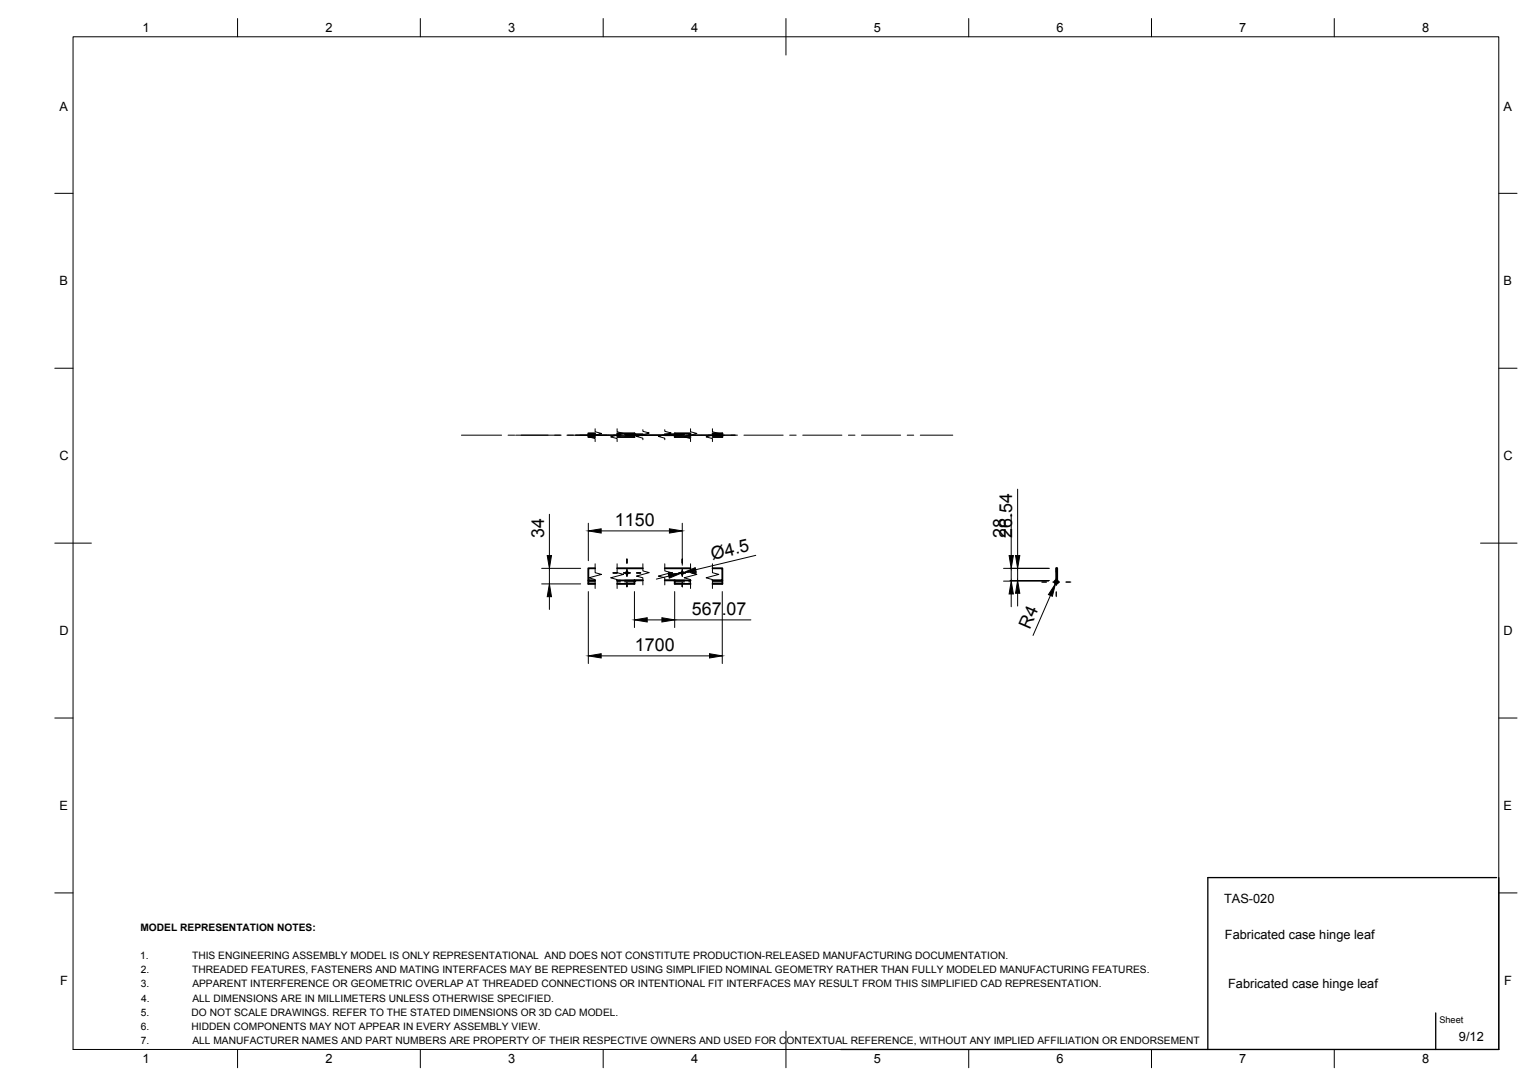
ISO-10303-21;
HEADER;
/* Generated by software containing ST-Developer
 * from STEP Tools, Inc. (www.steptools.com) 
 */

FILE_DESCRIPTION(
/* description */ (''),
/* implementation_level */ '2;1');

FILE_NAME(
/* name */ 'Fabricated case hinge leaf.step',
/* time_stamp */ '2026-11-15T17:46:57-08:00',
/* author */ (''),
/* organization */ (''),
/* preprocessor_version */ 'ST-DEVELOPER v20.2',
/* originating_system */ 'Autodesk Translation Framework v15.17.0.0',
/* authorisation */ '');

FILE_SCHEMA (('AUTOMOTIVE_DESIGN { 1 0 10303 214 3 1 1 }'));
ENDSEC;

DATA;
#10=MECHANICAL_DESIGN_GEOMETRIC_PRESENTATION_REPRESENTATION('',(#381),#12963);
#357=SHAPE_REPRESENTATION_RELATIONSHIP('SRR','None',#13041,#369);
#369=ADVANCED_BREP_SHAPE_REPRESENTATION('',(#393),#12957);
#381=STYLED_ITEM('',(#13110),#393);
#393=MANIFOLD_SOLID_BREP('Body1',#4815);
#423=FACE_BOUND('',#962,.T.);
#424=FACE_BOUND('',#963,.T.);
#425=FACE_BOUND('',#970,.T.);
#426=FACE_BOUND('',#972,.T.);
#427=FACE_BOUND('',#973,.T.);
#428=FACE_BOUND('',#979,.T.);
#527=PLANE('',#5108);
#528=PLANE('',#5112);
#529=PLANE('',#5113);
#530=PLANE('',#5114);
#531=PLANE('',#5115);
#532=PLANE('',#5116);
#533=PLANE('',#5123);
#534=PLANE('',#5124);
#535=PLANE('',#5131);
#536=PLANE('',#5132);
#537=PLANE('',#5133);
#676=FACE_OUTER_BOUND('',#956,.T.);
#677=FACE_OUTER_BOUND('',#957,.T.);
#678=FACE_OUTER_BOUND('',#958,.T.);
#679=FACE_OUTER_BOUND('',#959,.T.);
#680=FACE_OUTER_BOUND('',#960,.T.);
#681=FACE_OUTER_BOUND('',#961,.T.);
#682=FACE_OUTER_BOUND('',#964,.T.);
#683=FACE_OUTER_BOUND('',#965,.T.);
#684=FACE_OUTER_BOUND('',#966,.T.);
#685=FACE_OUTER_BOUND('',#967,.T.);
#686=FACE_OUTER_BOUND('',#968,.T.);
#687=FACE_OUTER_BOUND('',#969,.T.);
#688=FACE_OUTER_BOUND('',#971,.T.);
#689=FACE_OUTER_BOUND('',#974,.T.);
#690=FACE_OUTER_BOUND('',#975,.T.);
#691=FACE_OUTER_BOUND('',#976,.T.);
#692=FACE_OUTER_BOUND('',#977,.T.);
#693=FACE_OUTER_BOUND('',#978,.T.);
#956=EDGE_LOOP('',(#3604,#3605,#3606,#3607));
#957=EDGE_LOOP('',(#3608,#3609,#3610,#3611));
#958=EDGE_LOOP('',(#3612,#3613,#3614,#3615));
#959=EDGE_LOOP('',(#3616,#3617,#3618,#3619));
#960=EDGE_LOOP('',(#3620,#3621,#3622,#3623));
#961=EDGE_LOOP('',(#3624,#3625,#3626,#3627,#3628,#3629,#3630,#3631,#3632,
#3633,#3634,#3635));
#962=EDGE_LOOP('',(#3636));
#963=EDGE_LOOP('',(#3637));
#964=EDGE_LOOP('',(#3638,#3639,#3640,#3641,#3642,#3643));
#965=EDGE_LOOP('',(#3644,#3645,#3646,#3647,#3648,#3649));
#966=EDGE_LOOP('',(#3650,#3651,#3652,#3653,#3654));
#967=EDGE_LOOP('',(#3655,#3656,#3657,#3658));
#968=EDGE_LOOP('',(#3659,#3660,#3661,#3662));
#969=EDGE_LOOP('',(#3663,#3664,#3665,#3666));
#970=EDGE_LOOP('',(#3667,#3668,#3669));
#971=EDGE_LOOP('',(#3670,#3671,#3672,#3673,#3674,#3675,#3676,#3677,#3678,
#3679,#3680,#3681,#3682,#3683,#3684,#3685));
#972=EDGE_LOOP('',(#3686));
#973=EDGE_LOOP('',(#3687));
#974=EDGE_LOOP('',(#3688,#3689,#3690,#3691));
#975=EDGE_LOOP('',(#3692,#3693,#3694,#3695));
#976=EDGE_LOOP('',(#3696,#3697,#3698,#3699,#3700));
#977=EDGE_LOOP('',(#3701,#3702,#3703,#3704));
#978=EDGE_LOOP('',(#3705,#3706,#3707,#3708));
#979=EDGE_LOOP('',(#3709,#3710,#3711));
#1336=LINE('',#7043,#1738);
#1337=LINE('',#7049,#1739);
#1338=LINE('',#7054,#1740);
#1339=LINE('',#7058,#1741);
#1340=LINE('',#7059,#1742);
#1341=LINE('',#7062,#1743);
#1342=LINE('',#7065,#1744);
#1343=LINE('',#7068,#1745);
#1344=LINE('',#7070,#1746);
#1345=LINE('',#7071,#1747);
#1346=LINE('',#7074,#1748);
#1347=LINE('',#7076,#1749);
#1348=LINE('',#7078,#1750);
#1349=LINE('',#7080,#1751);
#1350=LINE('',#7082,#1752);
#1351=LINE('',#7084,#1753);
#1352=LINE('',#7086,#1754);
#1353=LINE('',#7088,#1755);
#1354=LINE('',#7089,#1756);
#1355=LINE('',#7092,#1757);
#1356=LINE('',#7094,#1758);
#1357=LINE('',#7096,#1759);
#1358=LINE('',#7097,#1760);
#1359=LINE('',#7100,#1761);
#1360=LINE('',#7102,#1762);
#1361=LINE('',#7104,#1763);
#1362=LINE('',#7105,#1764);
#1363=LINE('',#7110,#1765);
#1364=LINE('',#7115,#1766);
#1365=LINE('',#7118,#1767);
#1366=LINE('',#7122,#1768);
#1367=LINE('',#7123,#1769);
#1368=LINE('',#7124,#1770);
#1369=LINE('',#7127,#1771);
#1370=LINE('',#7129,#1772);
#1371=LINE('',#7131,#1773);
#1372=LINE('',#7133,#1774);
#1373=LINE('',#7135,#1775);
#1374=LINE('',#7136,#1776);
#1375=LINE('',#7145,#1777);
#1738=VECTOR('',#5851,0.225000000000001);
#1739=VECTOR('',#5858,0.224999999999994);
#1740=VECTOR('',#5863,1.);
#1741=VECTOR('',#5866,1.);
#1742=VECTOR('',#5867,1.);
#1743=VECTOR('',#5870,1.);
#1744=VECTOR('',#5873,1.);
#1745=VECTOR('',#5876,1.);
#1746=VECTOR('',#5877,1.);
#1747=VECTOR('',#5878,1.);
#1748=VECTOR('',#5881,1.);
#1749=VECTOR('',#5882,1.);
#1750=VECTOR('',#5883,1.);
#1751=VECTOR('',#5884,1.);
#1752=VECTOR('',#5885,1.);
#1753=VECTOR('',#5886,1.);
#1754=VECTOR('',#5887,1.);
#1755=VECTOR('',#5888,1.);
#1756=VECTOR('',#5889,1.);
#1757=VECTOR('',#5892,1.);
#1758=VECTOR('',#5893,1.);
#1759=VECTOR('',#5894,1.);
#1760=VECTOR('',#5895,1.);
#1761=VECTOR('',#5898,1.);
#1762=VECTOR('',#5899,1.);
#1763=VECTOR('',#5900,1.);
#1764=VECTOR('',#5901,1.);
#1765=VECTOR('',#5906,1.);
#1766=VECTOR('',#5913,1.);
#1767=VECTOR('',#5916,1.);
#1768=VECTOR('',#5921,1.);
#1769=VECTOR('',#5922,1.);
#1770=VECTOR('',#5923,1.);
#1771=VECTOR('',#5926,1.);
#1772=VECTOR('',#5927,1.);
#1773=VECTOR('',#5928,1.);
#1774=VECTOR('',#5929,1.);
#1775=VECTOR('',#5930,1.);
#1776=VECTOR('',#5931,1.);
#1777=VECTOR('',#5948,1.);
#1966=CIRCLE('',#5103,0.225000000000001);
#1967=CIRCLE('',#5104,0.225000000000001);
#1968=CIRCLE('',#5106,0.224999999999994);
#1969=CIRCLE('',#5107,0.224999999999994);
#1970=CIRCLE('',#5109,0.42);
#1971=CIRCLE('',#5111,0.42);
#1972=CIRCLE('',#5117,0.4);
#1973=CIRCLE('',#5118,0.22);
#1974=CIRCLE('',#5120,0.4);
#1975=CIRCLE('',#5122,0.22);
#1976=CIRCLE('',#5126,0.22);
#1977=CIRCLE('',#5127,0.22);
#1978=CIRCLE('',#5129,0.4);
#1979=CIRCLE('',#5130,0.4);
#2176=VERTEX_POINT('',#7040);
#2177=VERTEX_POINT('',#7042);
#2178=VERTEX_POINT('',#7046);
#2179=VERTEX_POINT('',#7048);
#2180=VERTEX_POINT('',#7052);
#2181=VERTEX_POINT('',#7053);
#2182=VERTEX_POINT('',#7055);
#2183=VERTEX_POINT('',#7057);
#2184=VERTEX_POINT('',#7061);
#2185=VERTEX_POINT('',#7063);
#2186=VERTEX_POINT('',#7067);
#2187=VERTEX_POINT('',#7069);
#2188=VERTEX_POINT('',#7073);
#2189=VERTEX_POINT('',#7075);
#2190=VERTEX_POINT('',#7077);
#2191=VERTEX_POINT('',#7079);
#2192=VERTEX_POINT('',#7081);
#2193=VERTEX_POINT('',#7083);
#2194=VERTEX_POINT('',#7085);
#2195=VERTEX_POINT('',#7087);
#2196=VERTEX_POINT('',#7091);
#2197=VERTEX_POINT('',#7093);
#2198=VERTEX_POINT('',#7095);
#2199=VERTEX_POINT('',#7099);
#2200=VERTEX_POINT('',#7101);
#2201=VERTEX_POINT('',#7103);
#2202=VERTEX_POINT('',#7107);
#2203=VERTEX_POINT('',#7109);
#2204=VERTEX_POINT('',#7113);
#2205=VERTEX_POINT('',#7117);
#2206=VERTEX_POINT('',#7121);
#2207=VERTEX_POINT('',#7126);
#2208=VERTEX_POINT('',#7128);
#2209=VERTEX_POINT('',#7130);
#2210=VERTEX_POINT('',#7132);
#2211=VERTEX_POINT('',#7134);
#2698=EDGE_CURVE('',#2176,#2176,#1966,.T.);
#2699=EDGE_CURVE('',#2176,#2177,#1336,.T.);
#2700=EDGE_CURVE('',#2177,#2177,#1967,.T.);
#2701=EDGE_CURVE('',#2178,#2178,#1968,.T.);
#2702=EDGE_CURVE('',#2178,#2179,#1337,.T.);
#2703=EDGE_CURVE('',#2179,#2179,#1969,.T.);
#2704=EDGE_CURVE('',#2180,#2181,#1338,.T.);
#2705=EDGE_CURVE('',#2182,#2180,#1970,.T.);
#2706=EDGE_CURVE('',#2183,#2182,#1339,.T.);
#2707=EDGE_CURVE('',#2181,#2183,#1340,.T.);
#2708=EDGE_CURVE('',#2184,#2180,#1341,.T.);
#2709=EDGE_CURVE('',#2185,#2184,#1971,.T.);
#2710=EDGE_CURVE('',#2182,#2185,#1342,.T.);
#2711=EDGE_CURVE('',#2186,#2184,#1343,.T.);
#2712=EDGE_CURVE('',#2187,#2186,#1344,.T.);
#2713=EDGE_CURVE('',#2185,#2187,#1345,.T.);
#2714=EDGE_CURVE('',#2188,#2187,#1346,.T.);
#2715=EDGE_CURVE('',#2188,#2189,#1347,.T.);
#2716=EDGE_CURVE('',#2189,#2190,#1348,.T.);
#2717=EDGE_CURVE('',#2190,#2191,#1349,.T.);
#2718=EDGE_CURVE('',#2191,#2192,#1350,.T.);
#2719=EDGE_CURVE('',#2193,#2192,#1351,.T.);
#2720=EDGE_CURVE('',#2193,#2194,#1352,.T.);
#2721=EDGE_CURVE('',#2194,#2195,#1353,.T.);
#2722=EDGE_CURVE('',#2183,#2195,#1354,.T.);
#2723=EDGE_CURVE('',#2196,#2186,#1355,.T.);
#2724=EDGE_CURVE('',#2196,#2197,#1356,.T.);
#2725=EDGE_CURVE('',#2197,#2198,#1357,.T.);
#2726=EDGE_CURVE('',#2198,#2188,#1358,.T.);
#2727=EDGE_CURVE('',#2195,#2199,#1359,.T.);
#2728=EDGE_CURVE('',#2199,#2200,#1360,.T.);
#2729=EDGE_CURVE('',#2201,#2200,#1361,.T.);
#2730=EDGE_CURVE('',#2181,#2201,#1362,.T.);
#2731=EDGE_CURVE('',#2202,#2194,#1972,.T.);
#2732=EDGE_CURVE('',#2203,#2202,#1363,.T.);
#2733=EDGE_CURVE('',#2199,#2203,#1973,.T.);
#2734=EDGE_CURVE('',#2204,#2193,#1974,.T.);
#2735=EDGE_CURVE('',#2202,#2204,#1364,.T.);
#2736=EDGE_CURVE('',#2205,#2203,#1365,.T.);
#2737=EDGE_CURVE('',#2200,#2205,#1975,.T.);
#2738=EDGE_CURVE('',#2192,#2206,#1366,.T.);
#2739=EDGE_CURVE('',#2206,#2204,#1367,.T.);
#2740=EDGE_CURVE('',#2205,#2201,#1368,.T.);
#2741=EDGE_CURVE('',#2207,#2206,#1369,.T.);
#2742=EDGE_CURVE('',#2207,#2208,#1370,.T.);
#2743=EDGE_CURVE('',#2208,#2209,#1371,.T.);
#2744=EDGE_CURVE('',#2209,#2210,#1372,.T.);
#2745=EDGE_CURVE('',#2210,#2211,#1373,.T.);
#2746=EDGE_CURVE('',#2211,#2196,#1374,.T.);
#2747=EDGE_CURVE('',#2197,#2211,#1976,.T.);
#2748=EDGE_CURVE('',#2198,#2210,#1977,.T.);
#2749=EDGE_CURVE('',#2209,#2189,#1978,.T.);
#2750=EDGE_CURVE('',#2208,#2190,#1979,.T.);
#2751=EDGE_CURVE('',#2191,#2207,#1375,.T.);
#3604=ORIENTED_EDGE('',*,*,#2698,.F.);
#3605=ORIENTED_EDGE('',*,*,#2699,.T.);
#3606=ORIENTED_EDGE('',*,*,#2700,.F.);
#3607=ORIENTED_EDGE('',*,*,#2699,.F.);
#3608=ORIENTED_EDGE('',*,*,#2701,.F.);
#3609=ORIENTED_EDGE('',*,*,#2702,.T.);
#3610=ORIENTED_EDGE('',*,*,#2703,.F.);
#3611=ORIENTED_EDGE('',*,*,#2702,.F.);
#3612=ORIENTED_EDGE('',*,*,#2704,.F.);
#3613=ORIENTED_EDGE('',*,*,#2705,.F.);
#3614=ORIENTED_EDGE('',*,*,#2706,.F.);
#3615=ORIENTED_EDGE('',*,*,#2707,.F.);
#3616=ORIENTED_EDGE('',*,*,#2708,.F.);
#3617=ORIENTED_EDGE('',*,*,#2709,.F.);
#3618=ORIENTED_EDGE('',*,*,#2710,.F.);
#3619=ORIENTED_EDGE('',*,*,#2705,.T.);
#3620=ORIENTED_EDGE('',*,*,#2711,.F.);
#3621=ORIENTED_EDGE('',*,*,#2712,.F.);
#3622=ORIENTED_EDGE('',*,*,#2713,.F.);
#3623=ORIENTED_EDGE('',*,*,#2709,.T.);
#3624=ORIENTED_EDGE('',*,*,#2706,.T.);
#3625=ORIENTED_EDGE('',*,*,#2710,.T.);
#3626=ORIENTED_EDGE('',*,*,#2713,.T.);
#3627=ORIENTED_EDGE('',*,*,#2714,.F.);
#3628=ORIENTED_EDGE('',*,*,#2715,.T.);
#3629=ORIENTED_EDGE('',*,*,#2716,.T.);
#3630=ORIENTED_EDGE('',*,*,#2717,.T.);
#3631=ORIENTED_EDGE('',*,*,#2718,.T.);
#3632=ORIENTED_EDGE('',*,*,#2719,.F.);
#3633=ORIENTED_EDGE('',*,*,#2720,.T.);
#3634=ORIENTED_EDGE('',*,*,#2721,.T.);
#3635=ORIENTED_EDGE('',*,*,#2722,.F.);
#3636=ORIENTED_EDGE('',*,*,#2700,.T.);
#3637=ORIENTED_EDGE('',*,*,#2703,.T.);
#3638=ORIENTED_EDGE('',*,*,#2712,.T.);
#3639=ORIENTED_EDGE('',*,*,#2723,.F.);
#3640=ORIENTED_EDGE('',*,*,#2724,.T.);
#3641=ORIENTED_EDGE('',*,*,#2725,.T.);
#3642=ORIENTED_EDGE('',*,*,#2726,.T.);
#3643=ORIENTED_EDGE('',*,*,#2714,.T.);
#3644=ORIENTED_EDGE('',*,*,#2707,.T.);
#3645=ORIENTED_EDGE('',*,*,#2722,.T.);
#3646=ORIENTED_EDGE('',*,*,#2727,.T.);
#3647=ORIENTED_EDGE('',*,*,#2728,.T.);
#3648=ORIENTED_EDGE('',*,*,#2729,.F.);
#3649=ORIENTED_EDGE('',*,*,#2730,.F.);
#3650=ORIENTED_EDGE('',*,*,#2727,.F.);
#3651=ORIENTED_EDGE('',*,*,#2721,.F.);
#3652=ORIENTED_EDGE('',*,*,#2731,.F.);
#3653=ORIENTED_EDGE('',*,*,#2732,.F.);
#3654=ORIENTED_EDGE('',*,*,#2733,.F.);
#3655=ORIENTED_EDGE('',*,*,#2720,.F.);
#3656=ORIENTED_EDGE('',*,*,#2734,.F.);
#3657=ORIENTED_EDGE('',*,*,#2735,.F.);
#3658=ORIENTED_EDGE('',*,*,#2731,.T.);
#3659=ORIENTED_EDGE('',*,*,#2728,.F.);
#3660=ORIENTED_EDGE('',*,*,#2733,.T.);
#3661=ORIENTED_EDGE('',*,*,#2736,.F.);
#3662=ORIENTED_EDGE('',*,*,#2737,.F.);
#3663=ORIENTED_EDGE('',*,*,#2719,.T.);
#3664=ORIENTED_EDGE('',*,*,#2738,.T.);
#3665=ORIENTED_EDGE('',*,*,#2739,.T.);
#3666=ORIENTED_EDGE('',*,*,#2734,.T.);
#3667=ORIENTED_EDGE('',*,*,#2737,.T.);
#3668=ORIENTED_EDGE('',*,*,#2740,.T.);
#3669=ORIENTED_EDGE('',*,*,#2729,.T.);
#3670=ORIENTED_EDGE('',*,*,#2704,.T.);
#3671=ORIENTED_EDGE('',*,*,#2730,.T.);
#3672=ORIENTED_EDGE('',*,*,#2740,.F.);
#3673=ORIENTED_EDGE('',*,*,#2736,.T.);
#3674=ORIENTED_EDGE('',*,*,#2732,.T.);
#3675=ORIENTED_EDGE('',*,*,#2735,.T.);
#3676=ORIENTED_EDGE('',*,*,#2739,.F.);
#3677=ORIENTED_EDGE('',*,*,#2741,.F.);
#3678=ORIENTED_EDGE('',*,*,#2742,.T.);
#3679=ORIENTED_EDGE('',*,*,#2743,.T.);
#3680=ORIENTED_EDGE('',*,*,#2744,.T.);
#3681=ORIENTED_EDGE('',*,*,#2745,.T.);
#3682=ORIENTED_EDGE('',*,*,#2746,.T.);
#3683=ORIENTED_EDGE('',*,*,#2723,.T.);
#3684=ORIENTED_EDGE('',*,*,#2711,.T.);
#3685=ORIENTED_EDGE('',*,*,#2708,.T.);
#3686=ORIENTED_EDGE('',*,*,#2698,.T.);
#3687=ORIENTED_EDGE('',*,*,#2701,.T.);
#3688=ORIENTED_EDGE('',*,*,#2725,.F.);
#3689=ORIENTED_EDGE('',*,*,#2747,.T.);
#3690=ORIENTED_EDGE('',*,*,#2745,.F.);
#3691=ORIENTED_EDGE('',*,*,#2748,.F.);
#3692=ORIENTED_EDGE('',*,*,#2716,.F.);
#3693=ORIENTED_EDGE('',*,*,#2749,.F.);
#3694=ORIENTED_EDGE('',*,*,#2743,.F.);
#3695=ORIENTED_EDGE('',*,*,#2750,.T.);
#3696=ORIENTED_EDGE('',*,*,#2726,.F.);
#3697=ORIENTED_EDGE('',*,*,#2748,.T.);
#3698=ORIENTED_EDGE('',*,*,#2744,.F.);
#3699=ORIENTED_EDGE('',*,*,#2749,.T.);
#3700=ORIENTED_EDGE('',*,*,#2715,.F.);
#3701=ORIENTED_EDGE('',*,*,#2751,.T.);
#3702=ORIENTED_EDGE('',*,*,#2741,.T.);
#3703=ORIENTED_EDGE('',*,*,#2738,.F.);
#3704=ORIENTED_EDGE('',*,*,#2718,.F.);
#3705=ORIENTED_EDGE('',*,*,#2750,.F.);
#3706=ORIENTED_EDGE('',*,*,#2742,.F.);
#3707=ORIENTED_EDGE('',*,*,#2751,.F.);
#3708=ORIENTED_EDGE('',*,*,#2717,.F.);
#3709=ORIENTED_EDGE('',*,*,#2724,.F.);
#3710=ORIENTED_EDGE('',*,*,#2746,.F.);
#3711=ORIENTED_EDGE('',*,*,#2747,.F.);
#4450=CYLINDRICAL_SURFACE('',#5102,0.225000000000001);
#4451=CYLINDRICAL_SURFACE('',#5105,0.224999999999994);
#4452=CYLINDRICAL_SURFACE('',#5110,0.42);
#4453=CYLINDRICAL_SURFACE('',#5119,0.4);
#4454=CYLINDRICAL_SURFACE('',#5121,0.22);
#4455=CYLINDRICAL_SURFACE('',#5125,0.22);
#4456=CYLINDRICAL_SURFACE('',#5128,0.4);
#4657=ADVANCED_FACE('',(#676),#4450,.F.);
#4658=ADVANCED_FACE('',(#677),#4451,.F.);
#4659=ADVANCED_FACE('',(#678),#527,.F.);
#4660=ADVANCED_FACE('',(#679),#4452,.F.);
#4661=ADVANCED_FACE('',(#680),#528,.T.);
#4662=ADVANCED_FACE('',(#681,#423,#424),#529,.T.);
#4663=ADVANCED_FACE('',(#682),#530,.T.);
#4664=ADVANCED_FACE('',(#683),#531,.T.);
#4665=ADVANCED_FACE('',(#684),#532,.F.);
#4666=ADVANCED_FACE('',(#685),#4453,.T.);
#4667=ADVANCED_FACE('',(#686),#4454,.F.);
#4668=ADVANCED_FACE('',(#687,#425),#533,.T.);
#4669=ADVANCED_FACE('',(#688,#426,#427),#534,.T.);
#4670=ADVANCED_FACE('',(#689),#4455,.F.);
#4671=ADVANCED_FACE('',(#690),#4456,.T.);
#4672=ADVANCED_FACE('',(#691),#535,.T.);
#4673=ADVANCED_FACE('',(#692),#536,.T.);
#4674=ADVANCED_FACE('',(#693,#428),#537,.F.);
#4815=CLOSED_SHELL('',(#4657,#4658,#4659,#4660,#4661,#4662,#4663,#4664,
#4665,#4666,#4667,#4668,#4669,#4670,#4671,#4672,#4673,#4674));
#5101=AXIS2_PLACEMENT_3D('',#7038,#5845,#5846);
#5102=AXIS2_PLACEMENT_3D('',#7039,#5847,#5848);
#5103=AXIS2_PLACEMENT_3D('',#7041,#5849,#5850);
#5104=AXIS2_PLACEMENT_3D('',#7044,#5852,#5853);
#5105=AXIS2_PLACEMENT_3D('',#7045,#5854,#5855);
#5106=AXIS2_PLACEMENT_3D('',#7047,#5856,#5857);
#5107=AXIS2_PLACEMENT_3D('',#7050,#5859,#5860);
#5108=AXIS2_PLACEMENT_3D('',#7051,#5861,#5862);
#5109=AXIS2_PLACEMENT_3D('',#7056,#5864,#5865);
#5110=AXIS2_PLACEMENT_3D('',#7060,#5868,#5869);
#5111=AXIS2_PLACEMENT_3D('',#7064,#5871,#5872);
#5112=AXIS2_PLACEMENT_3D('',#7066,#5874,#5875);
#5113=AXIS2_PLACEMENT_3D('',#7072,#5879,#5880);
#5114=AXIS2_PLACEMENT_3D('',#7090,#5890,#5891);
#5115=AXIS2_PLACEMENT_3D('',#7098,#5896,#5897);
#5116=AXIS2_PLACEMENT_3D('',#7106,#5902,#5903);
#5117=AXIS2_PLACEMENT_3D('',#7108,#5904,#5905);
#5118=AXIS2_PLACEMENT_3D('',#7111,#5907,#5908);
#5119=AXIS2_PLACEMENT_3D('',#7112,#5909,#5910);
#5120=AXIS2_PLACEMENT_3D('',#7114,#5911,#5912);
#5121=AXIS2_PLACEMENT_3D('',#7116,#5914,#5915);
#5122=AXIS2_PLACEMENT_3D('',#7119,#5917,#5918);
#5123=AXIS2_PLACEMENT_3D('',#7120,#5919,#5920);
#5124=AXIS2_PLACEMENT_3D('',#7125,#5924,#5925);
#5125=AXIS2_PLACEMENT_3D('',#7137,#5932,#5933);
#5126=AXIS2_PLACEMENT_3D('',#7138,#5934,#5935);
#5127=AXIS2_PLACEMENT_3D('',#7139,#5936,#5937);
#5128=AXIS2_PLACEMENT_3D('',#7140,#5938,#5939);
#5129=AXIS2_PLACEMENT_3D('',#7141,#5940,#5941);
#5130=AXIS2_PLACEMENT_3D('',#7142,#5942,#5943);
#5131=AXIS2_PLACEMENT_3D('',#7143,#5944,#5945);
#5132=AXIS2_PLACEMENT_3D('',#7144,#5946,#5947);
#5133=AXIS2_PLACEMENT_3D('',#7146,#5949,#5950);
#5845=DIRECTION('axis',(0.,0.,1.));
#5846=DIRECTION('refdir',(1.,0.,0.));
#5847=DIRECTION('center_axis',(1.,0.,0.));
#5848=DIRECTION('ref_axis',(0.,0.,-1.));
#5849=DIRECTION('center_axis',(1.,0.,0.));
#5850=DIRECTION('ref_axis',(0.,0.,-1.));
#5851=DIRECTION('',(1.,0.,0.));
#5852=DIRECTION('center_axis',(-1.,0.,0.));
#5853=DIRECTION('ref_axis',(0.,0.,-1.));
#5854=DIRECTION('center_axis',(1.,0.,0.));
#5855=DIRECTION('ref_axis',(0.,0.,-1.));
#5856=DIRECTION('center_axis',(1.,0.,0.));
#5857=DIRECTION('ref_axis',(0.,0.,-1.));
#5858=DIRECTION('',(1.,0.,0.));
#5859=DIRECTION('center_axis',(-1.,0.,0.));
#5860=DIRECTION('ref_axis',(0.,0.,-1.));
#5861=DIRECTION('center_axis',(0.,0.,1.));
#5862=DIRECTION('ref_axis',(1.,0.,0.));
#5863=DIRECTION('',(0.,-1.,0.));
#5864=DIRECTION('center_axis',(0.,0.,1.));
#5865=DIRECTION('ref_axis',(1.,0.,0.));
#5866=DIRECTION('',(0.,1.,0.));
#5867=DIRECTION('',(1.,0.,0.));
#5868=DIRECTION('center_axis',(0.,0.,1.));
#5869=DIRECTION('ref_axis',(1.,0.,0.));
#5870=DIRECTION('',(0.,0.,1.));
#5871=DIRECTION('center_axis',(0.,0.,1.));
#5872=DIRECTION('ref_axis',(1.,0.,0.));
#5873=DIRECTION('',(0.,0.,-1.));
#5874=DIRECTION('center_axis',(0.,0.,1.));
#5875=DIRECTION('ref_axis',(1.,0.,0.));
#5876=DIRECTION('',(0.,1.,0.));
#5877=DIRECTION('',(-1.,0.,0.));
#5878=DIRECTION('',(0.,-1.,0.));
#5879=DIRECTION('center_axis',(1.,0.,0.));
#5880=DIRECTION('ref_axis',(0.,1.,0.));
#5881=DIRECTION('',(0.,0.,1.));
#5882=DIRECTION('',(0.,1.,0.));
#5883=DIRECTION('',(0.,0.,-1.));
#5884=DIRECTION('',(0.,1.,0.));
#5885=DIRECTION('',(0.,0.,1.));
#5886=DIRECTION('',(0.,1.,0.));
#5887=DIRECTION('',(0.,0.,-1.));
#5888=DIRECTION('',(0.,-1.,0.));
#5889=DIRECTION('',(0.,0.,1.));
#5890=DIRECTION('center_axis',(0.,-1.,0.));
#5891=DIRECTION('ref_axis',(1.,0.,0.));
#5892=DIRECTION('',(0.,0.,1.));
#5893=DIRECTION('',(1.,0.,0.));
#5894=DIRECTION('',(0.,0.,1.));
#5895=DIRECTION('',(1.,0.,0.));
#5896=DIRECTION('center_axis',(0.,-1.,0.));
#5897=DIRECTION('ref_axis',(1.,0.,0.));
#5898=DIRECTION('',(-1.,0.,0.));
#5899=DIRECTION('',(0.,0.,1.));
#5900=DIRECTION('',(1.,0.,0.));
#5901=DIRECTION('',(0.,0.,1.));
#5902=DIRECTION('center_axis',(0.,0.,1.));
#5903=DIRECTION('ref_axis',(1.,0.,0.));
#5904=DIRECTION('center_axis',(0.,0.,1.));
#5905=DIRECTION('ref_axis',(1.,0.,0.));
#5906=DIRECTION('',(0.,1.,0.));
#5907=DIRECTION('center_axis',(0.,0.,-1.));
#5908=DIRECTION('ref_axis',(1.,0.,0.));
#5909=DIRECTION('center_axis',(0.,0.,1.));
#5910=DIRECTION('ref_axis',(-0.25881904510252,-0.965925826289069,0.));
#5911=DIRECTION('center_axis',(0.,0.,1.));
#5912=DIRECTION('ref_axis',(1.,0.,0.));
#5913=DIRECTION('',(0.,0.,1.));
#5914=DIRECTION('center_axis',(0.,0.,1.));
#5915=DIRECTION('ref_axis',(-0.213200716355611,-0.977008420918394,0.));
#5916=DIRECTION('',(0.,0.,-1.));
#5917=DIRECTION('center_axis',(0.,0.,-1.));
#5918=DIRECTION('ref_axis',(1.,0.,0.));
#5919=DIRECTION('center_axis',(0.,0.,1.));
#5920=DIRECTION('ref_axis',(1.,0.,0.));
#5921=DIRECTION('',(-1.,0.,0.));
#5922=DIRECTION('',(0.,-1.,0.));
#5923=DIRECTION('',(0.,-1.,0.));
#5924=DIRECTION('center_axis',(-1.,0.,0.));
#5925=DIRECTION('ref_axis',(0.,-1.,0.));
#5926=DIRECTION('',(0.,0.,1.));
#5927=DIRECTION('',(0.,-1.,0.));
#5928=DIRECTION('',(0.,0.,1.));
#5929=DIRECTION('',(0.,-1.,0.));
#5930=DIRECTION('',(0.,0.,-1.));
#5931=DIRECTION('',(0.,-1.,0.));
#5932=DIRECTION('center_axis',(0.,0.,1.));
#5933=DIRECTION('ref_axis',(-0.213200716355611,-0.977008420918394,0.));
#5934=DIRECTION('center_axis',(0.,0.,-1.));
#5935=DIRECTION('ref_axis',(1.,0.,0.));
#5936=DIRECTION('center_axis',(0.,0.,-1.));
#5937=DIRECTION('ref_axis',(1.,0.,0.));
#5938=DIRECTION('center_axis',(0.,0.,1.));
#5939=DIRECTION('ref_axis',(-0.25881904510252,-0.965925826289069,0.));
#5940=DIRECTION('center_axis',(0.,0.,1.));
#5941=DIRECTION('ref_axis',(1.,0.,0.));
#5942=DIRECTION('center_axis',(0.,0.,1.));
#5943=DIRECTION('ref_axis',(1.,0.,0.));
#5944=DIRECTION('center_axis',(0.,0.,1.));
#5945=DIRECTION('ref_axis',(1.,0.,0.));
#5946=DIRECTION('center_axis',(0.,1.,0.));
#5947=DIRECTION('ref_axis',(-1.,0.,0.));
#5948=DIRECTION('',(-1.,0.,0.));
#5949=DIRECTION('center_axis',(0.,0.,1.));
#5950=DIRECTION('ref_axis',(1.,0.,0.));
#7038=CARTESIAN_POINT('',(0.,0.,0.));
#7039=CARTESIAN_POINT('Origin',(0.,2.,55.));
#7040=CARTESIAN_POINT('',(0.,2.,55.225));
#7041=CARTESIAN_POINT('Origin',(0.,2.,55.));
#7042=CARTESIAN_POINT('',(0.2,2.,55.225));
#7043=CARTESIAN_POINT('',(0.,2.,55.225));
#7044=CARTESIAN_POINT('Origin',(0.2,2.,55.));
#7045=CARTESIAN_POINT('Origin',(0.,2.,115.));
#7046=CARTESIAN_POINT('',(0.,2.,115.225));
#7047=CARTESIAN_POINT('Origin',(0.,2.,115.));
#7048=CARTESIAN_POINT('',(0.2,2.,115.225));
#7049=CARTESIAN_POINT('',(0.,2.,115.225));
#7050=CARTESIAN_POINT('Origin',(0.2,2.,115.));
#7051=CARTESIAN_POINT('Origin',(0.,0.,113.343333333333));
#7052=CARTESIAN_POINT('',(0.,0.42,113.343333333333));
#7053=CARTESIAN_POINT('',(0.,0.2,113.343333333333));
#7054=CARTESIAN_POINT('',(0.,1.5,113.343333333333));
#7055=CARTESIAN_POINT('',(0.2,0.369323706252388,113.343333333333));
#7056=CARTESIAN_POINT('Origin',(0.,0.,113.343333333333));
#7057=CARTESIAN_POINT('',(0.2,0.2,113.343333333333));
#7058=CARTESIAN_POINT('',(0.2,0.1,113.343333333333));
#7059=CARTESIAN_POINT('',(0.,0.2,113.343333333333));
#7060=CARTESIAN_POINT('Origin',(0.,0.,56.6566666666667));
#7061=CARTESIAN_POINT('',(0.,0.42,56.6566666666667));
#7062=CARTESIAN_POINT('',(0.,0.42,56.6566666666667));
#7063=CARTESIAN_POINT('',(0.2,0.369323706252388,56.6566666666667));
#7064=CARTESIAN_POINT('Origin',(0.,0.,56.6566666666667));
#7065=CARTESIAN_POINT('',(0.2,0.369323706252388,56.6566666666667));
#7066=CARTESIAN_POINT('Origin',(0.,0.,56.6566666666667));
#7067=CARTESIAN_POINT('',(0.,0.2,56.6566666666667));
#7068=CARTESIAN_POINT('',(0.,1.5,56.6566666666667));
#7069=CARTESIAN_POINT('',(0.2,0.2,56.6566666666667));
#7070=CARTESIAN_POINT('',(0.,0.2,56.6566666666667));
#7071=CARTESIAN_POINT('',(0.2,0.1,56.6566666666667));
#7072=CARTESIAN_POINT('Origin',(0.2,0.2,0.));
#7073=CARTESIAN_POINT('',(0.2,0.2,56.6466666666667));
#7074=CARTESIAN_POINT('',(0.2,0.2,0.));
#7075=CARTESIAN_POINT('',(0.2,0.346410161513776,56.6466666666667));
#7076=CARTESIAN_POINT('',(0.2,0.1,56.6466666666667));
#7077=CARTESIAN_POINT('',(0.2,0.346410161513776,0.));
#7078=CARTESIAN_POINT('',(0.2,0.346410161513776,0.));
#7079=CARTESIAN_POINT('',(0.2,3.,0.));
#7080=CARTESIAN_POINT('',(0.2,0.2,0.));
#7081=CARTESIAN_POINT('',(0.2,3.,170.));
#7082=CARTESIAN_POINT('',(0.2,3.,0.));
#7083=CARTESIAN_POINT('',(0.2,0.346410161513776,170.));
#7084=CARTESIAN_POINT('',(0.2,0.2,170.));
#7085=CARTESIAN_POINT('',(0.2,0.346410161513776,113.353333333333));
#7086=CARTESIAN_POINT('',(0.2,0.346410161513776,113.353333333333));
#7087=CARTESIAN_POINT('',(0.2,0.2,113.353333333333));
#7088=CARTESIAN_POINT('',(0.2,0.1,113.353333333333));
#7089=CARTESIAN_POINT('',(0.2,0.2,0.));
#7090=CARTESIAN_POINT('Origin',(0.,0.2,0.));
#7091=CARTESIAN_POINT('',(0.,0.2,0.));
#7092=CARTESIAN_POINT('',(0.,0.2,0.));
#7093=CARTESIAN_POINT('',(0.0916515138991168,0.2,0.));
#7094=CARTESIAN_POINT('',(0.,0.2,0.));
#7095=CARTESIAN_POINT('',(0.0916515138991168,0.2,56.6466666666667));
#7096=CARTESIAN_POINT('',(0.0916515138991168,0.2,0.));
#7097=CARTESIAN_POINT('',(0.,0.2,56.6466666666667));
#7098=CARTESIAN_POINT('Origin',(0.,0.2,0.));
#7099=CARTESIAN_POINT('',(0.0916515138991168,0.2,113.353333333333));
#7100=CARTESIAN_POINT('',(0.,0.2,113.353333333333));
#7101=CARTESIAN_POINT('',(0.0916515138991168,0.2,170.));
#7102=CARTESIAN_POINT('',(0.0916515138991168,0.2,113.353333333333));
#7103=CARTESIAN_POINT('',(0.,0.2,170.));
#7104=CARTESIAN_POINT('',(0.,0.2,170.));
#7105=CARTESIAN_POINT('',(0.,0.2,0.));
#7106=CARTESIAN_POINT('Origin',(0.,0.,113.353333333333));
#7107=CARTESIAN_POINT('',(0.,0.4,113.353333333333));
#7108=CARTESIAN_POINT('Origin',(0.,0.,113.353333333333));
#7109=CARTESIAN_POINT('',(0.,0.22,113.353333333333));
#7110=CARTESIAN_POINT('',(0.,1.5,113.353333333333));
#7111=CARTESIAN_POINT('Origin',(0.,0.,113.353333333333));
#7112=CARTESIAN_POINT('Origin',(0.,0.,113.353333333333));
#7113=CARTESIAN_POINT('',(0.,0.4,170.));
#7114=CARTESIAN_POINT('Origin',(0.,0.,170.));
#7115=CARTESIAN_POINT('',(0.,0.4,113.353333333333));
#7116=CARTESIAN_POINT('Origin',(0.,0.,113.353333333333));
#7117=CARTESIAN_POINT('',(0.,0.22,170.));
#7118=CARTESIAN_POINT('',(0.,0.22,113.353333333333));
#7119=CARTESIAN_POINT('Origin',(0.,0.,170.));
#7120=CARTESIAN_POINT('Origin',(0.1,1.6,170.));
#7121=CARTESIAN_POINT('',(0.,3.,170.));
#7122=CARTESIAN_POINT('',(0.2,3.,170.));
#7123=CARTESIAN_POINT('',(0.,3.,170.));
#7124=CARTESIAN_POINT('',(0.,3.,170.));
#7125=CARTESIAN_POINT('Origin',(0.,3.,0.));
#7126=CARTESIAN_POINT('',(0.,3.,0.));
#7127=CARTESIAN_POINT('',(0.,3.,0.));
#7128=CARTESIAN_POINT('',(0.,0.4,0.));
#7129=CARTESIAN_POINT('',(0.,3.,0.));
#7130=CARTESIAN_POINT('',(0.,0.4,56.6466666666667));
#7131=CARTESIAN_POINT('',(0.,0.4,0.));
#7132=CARTESIAN_POINT('',(0.,0.22,56.6466666666667));
#7133=CARTESIAN_POINT('',(0.,1.5,56.6466666666667));
#7134=CARTESIAN_POINT('',(0.,0.22,0.));
#7135=CARTESIAN_POINT('',(0.,0.22,0.));
#7136=CARTESIAN_POINT('',(0.,3.,0.));
#7137=CARTESIAN_POINT('Origin',(0.,0.,0.));
#7138=CARTESIAN_POINT('Origin',(0.,0.,0.));
#7139=CARTESIAN_POINT('Origin',(0.,0.,56.6466666666667));
#7140=CARTESIAN_POINT('Origin',(0.,0.,0.));
#7141=CARTESIAN_POINT('Origin',(0.,0.,56.6466666666667));
#7142=CARTESIAN_POINT('Origin',(0.,0.,0.));
#7143=CARTESIAN_POINT('Origin',(0.,0.,56.6466666666667));
#7144=CARTESIAN_POINT('Origin',(0.2,3.,0.));
#7145=CARTESIAN_POINT('',(0.2,3.,0.));
#7146=CARTESIAN_POINT('Origin',(0.1,1.6,0.));
#12943=UNCERTAINTY_MEASURE_WITH_UNIT(LENGTH_MEASURE(0.001),#12964,
'DISTANCE_ACCURACY_VALUE',
'Maximum model space distance between geometric entities at asserted c
onnectivities');
#12949=UNCERTAINTY_MEASURE_WITH_UNIT(LENGTH_MEASURE(0.001),#12964,
'DISTANCE_ACCURACY_VALUE',
'Maximum model space distance between geometric entities at asserted c
onnectivities');
#12957=(
GEOMETRIC_REPRESENTATION_CONTEXT(3)
GLOBAL_UNCERTAINTY_ASSIGNED_CONTEXT((#12943))
GLOBAL_UNIT_ASSIGNED_CONTEXT((#12964,#12966,#12967))
REPRESENTATION_CONTEXT('','3D')
);
#12963=(
GEOMETRIC_REPRESENTATION_CONTEXT(3)
GLOBAL_UNCERTAINTY_ASSIGNED_CONTEXT((#12949))
GLOBAL_UNIT_ASSIGNED_CONTEXT((#12964,#12966,#12967))
REPRESENTATION_CONTEXT('','3D')
);
#12964=(
LENGTH_UNIT()
NAMED_UNIT(*)
SI_UNIT(.CENTI.,.METRE.)
);
#12966=(
NAMED_UNIT(*)
PLANE_ANGLE_UNIT()
SI_UNIT($,.RADIAN.)
);
#12967=(
NAMED_UNIT(*)
SI_UNIT($,.STERADIAN.)
SOLID_ANGLE_UNIT()
);
#12975=SHAPE_DEFINITION_REPRESENTATION(#12988,#13041);
#12988=PRODUCT_DEFINITION_SHAPE('',$,#13055);
#13041=SHAPE_REPRESENTATION('',(#5101),#12957);
#13047=PRODUCT_DEFINITION_CONTEXT('part definition',#13088,'design');
#13055=PRODUCT_DEFINITION('Fabricated case hinge leaf',
'Fabricated case hinge leaf',#13068,#13047);
#13068=PRODUCT_DEFINITION_FORMATION('',$,#13097);
#13088=APPLICATION_CONTEXT(
'Core Data for Automotive Mechanical Design Process');
#13089=PRODUCT_CONTEXT('part definition',#13088,'mechanical');
#13097=PRODUCT('Fabricated case hinge leaf',
'Fabricated case hinge leaf',$,(#13089));
#13110=PRESENTATION_STYLE_ASSIGNMENT((#13123));
#13123=SURFACE_STYLE_USAGE(.BOTH.,#13136);
#13136=SURFACE_SIDE_STYLE('',(#13149));
#13149=SURFACE_STYLE_FILL_AREA(#13162);
#13162=FILL_AREA_STYLE('Fabricated case hinge leaf finish',(#13175));
#13175=FILL_AREA_STYLE_COLOUR('Fabricated case hinge leaf finish',#13188);
#13188=COLOUR_RGB('Fabricated case hinge leaf finish',0.607843137254902,
0.647058823529412,0.701960784313725);
ENDSEC;
END-ISO-10303-21;
